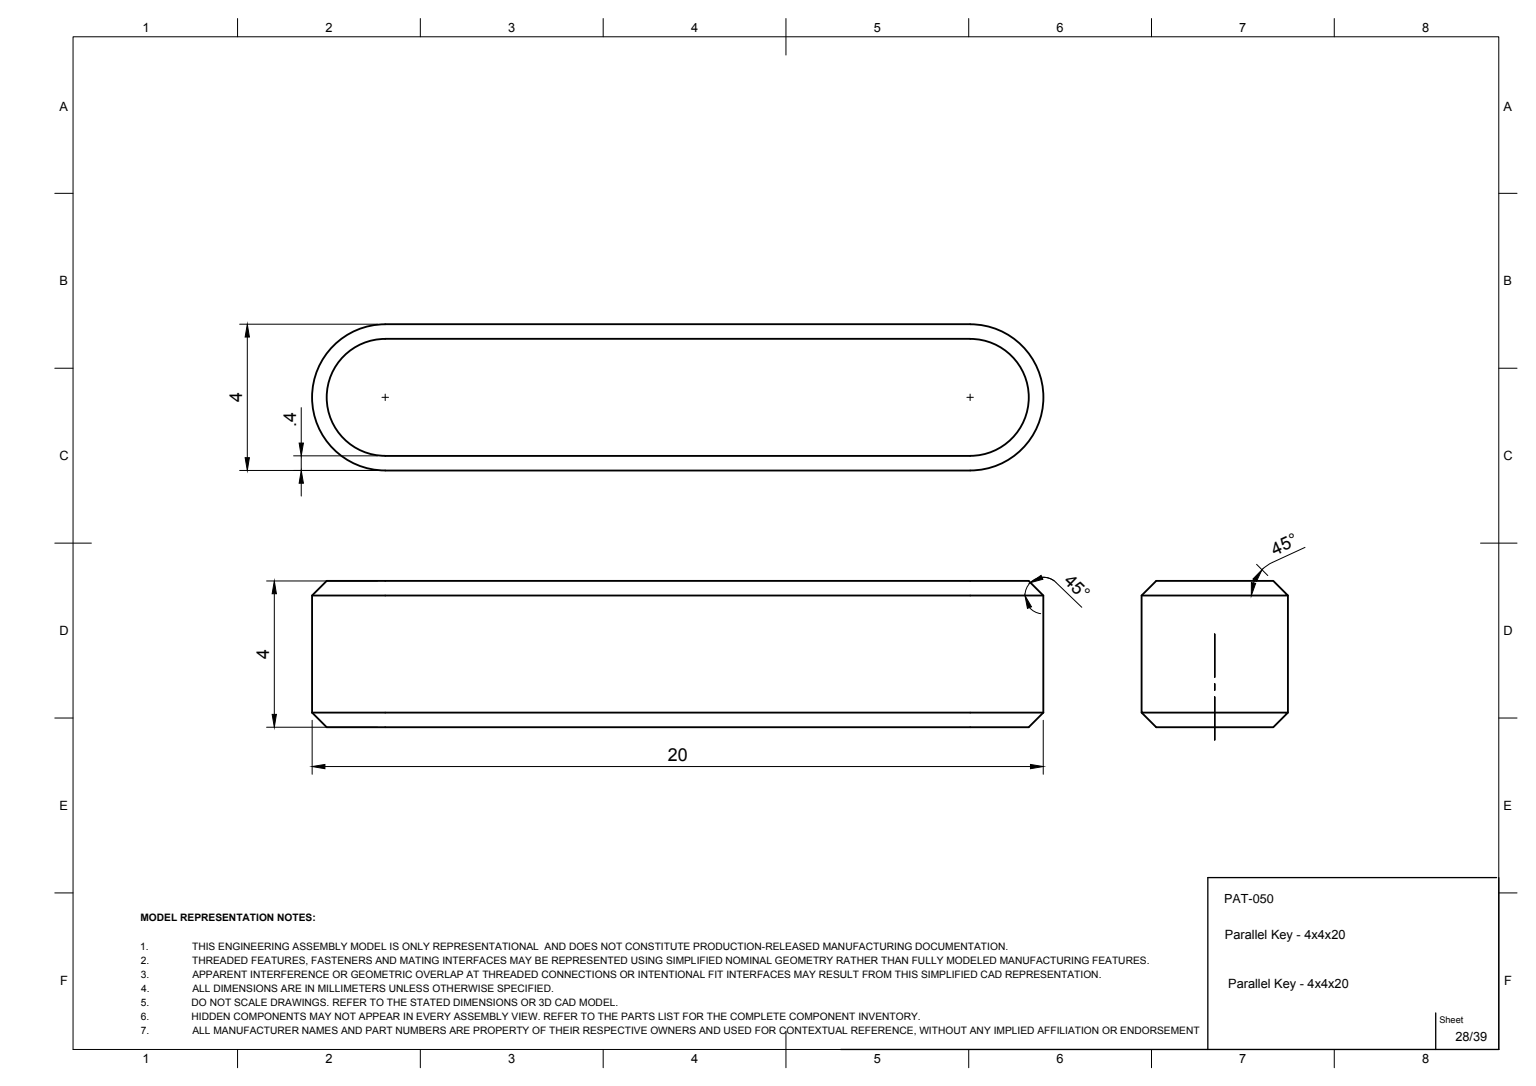
ISO-10303-21;
HEADER;
/* Generated by software containing ST-Developer
 * from STEP Tools, Inc. (www.steptools.com) 
 */

FILE_DESCRIPTION(
/* description */ ('Hand wheel with handle and shaft collar'),
/* implementation_level */ '2;1');

FILE_NAME(
/* name */ 'Parallel Key - 4x4x20.step',
/* time_stamp */ '2026-10-28T03:23:19-07:00',
/* author */ (''),
/* organization */ (''),
/* preprocessor_version */ 'ST-DEVELOPER v20.2',
/* originating_system */ 'Autodesk Translation Framework v15.17.0.0',
/* authorisation */ '');

FILE_SCHEMA (('AUTOMOTIVE_DESIGN { 1 0 10303 214 3 1 1 }'));
ENDSEC;

DATA;
#10=MECHANICAL_DESIGN_GEOMETRIC_PRESENTATION_REPRESENTATION('',(#423),#10510);
#308=CONICAL_SURFACE('',#6130,0.18,0.785398163397448);
#309=CONICAL_SURFACE('',#6134,0.18,0.785398163397448);
#310=CONICAL_SURFACE('',#6142,0.18,0.785398163397449);
#311=CONICAL_SURFACE('',#6145,0.18,0.785398163397449);
#352=SHAPE_REPRESENTATION_RELATIONSHIP('SRR','None',#10670,#384);
#384=ADVANCED_BREP_SHAPE_REPRESENTATION('',(#469),#10497);
#423=STYLED_ITEM('',(#10908),#469);
#469=MANIFOLD_SOLID_BREP('Body1',#5323);
#702=PLANE('',#6129);
#703=PLANE('',#6133);
#704=PLANE('',#6139);
#705=PLANE('',#6140);
#706=PLANE('',#6141);
#707=PLANE('',#6144);
#708=PLANE('',#6149);
#709=PLANE('',#6150);
#962=FACE_OUTER_BOUND('',#1376,.T.);
#963=FACE_OUTER_BOUND('',#1377,.T.);
#964=FACE_OUTER_BOUND('',#1378,.T.);
#965=FACE_OUTER_BOUND('',#1379,.T.);
#966=FACE_OUTER_BOUND('',#1380,.T.);
#967=FACE_OUTER_BOUND('',#1381,.T.);
#968=FACE_OUTER_BOUND('',#1382,.T.);
#969=FACE_OUTER_BOUND('',#1383,.T.);
#970=FACE_OUTER_BOUND('',#1384,.T.);
#971=FACE_OUTER_BOUND('',#1385,.T.);
#972=FACE_OUTER_BOUND('',#1386,.T.);
#973=FACE_OUTER_BOUND('',#1387,.T.);
#974=FACE_OUTER_BOUND('',#1388,.T.);
#975=FACE_OUTER_BOUND('',#1389,.T.);
#1376=EDGE_LOOP('',(#4407,#4408,#4409,#4410));
#1377=EDGE_LOOP('',(#4411,#4412,#4413,#4414));
#1378=EDGE_LOOP('',(#4415,#4416,#4417,#4418));
#1379=EDGE_LOOP('',(#4419,#4420,#4421,#4422));
#1380=EDGE_LOOP('',(#4423,#4424,#4425,#4426));
#1381=EDGE_LOOP('',(#4427,#4428,#4429,#4430));
#1382=EDGE_LOOP('',(#4431,#4432,#4433,#4434));
#1383=EDGE_LOOP('',(#4435,#4436,#4437,#4438));
#1384=EDGE_LOOP('',(#4439,#4440,#4441,#4442));
#1385=EDGE_LOOP('',(#4443,#4444,#4445,#4446));
#1386=EDGE_LOOP('',(#4447,#4448,#4449,#4450));
#1387=EDGE_LOOP('',(#4451,#4452,#4453,#4454));
#1388=EDGE_LOOP('',(#4455,#4456,#4457,#4458));
#1389=EDGE_LOOP('',(#4459,#4460,#4461,#4462));
#1714=LINE('',#9520,#2024);
#1715=LINE('',#9522,#2025);
#1716=LINE('',#9524,#2026);
#1717=LINE('',#9525,#2027);
#1718=LINE('',#9529,#2028);
#1719=LINE('',#9535,#2029);
#1720=LINE('',#9536,#2030);
#1721=LINE('',#9537,#2031);
#1722=LINE('',#9543,#2032);
#1723=LINE('',#9546,#2033);
#1724=LINE('',#9549,#2034);
#1725=LINE('',#9550,#2035);
#1726=LINE('',#9554,#2036);
#1727=LINE('',#9556,#2037);
#1728=LINE('',#9557,#2038);
#1729=LINE('',#9560,#2039);
#1730=LINE('',#9565,#2040);
#1731=LINE('',#9566,#2041);
#1732=LINE('',#9567,#2042);
#1733=LINE('',#9572,#2043);
#2024=VECTOR('',#7486,1.);
#2025=VECTOR('',#7487,1.);
#2026=VECTOR('',#7488,1.);
#2027=VECTOR('',#7489,1.);
#2028=VECTOR('',#7492,1.);
#2029=VECTOR('',#7499,1.);
#2030=VECTOR('',#7500,1.);
#2031=VECTOR('',#7501,1.);
#2032=VECTOR('',#7510,1.);
#2033=VECTOR('',#7513,1.);
#2034=VECTOR('',#7516,1.);
#2035=VECTOR('',#7517,1.);
#2036=VECTOR('',#7522,1.);
#2037=VECTOR('',#7523,1.);
#2038=VECTOR('',#7524,1.);
#2039=VECTOR('',#7527,1.);
#2040=VECTOR('',#7532,1.);
#2041=VECTOR('',#7533,1.);
#2042=VECTOR('',#7534,1.);
#2043=VECTOR('',#7543,1.);
#2335=CIRCLE('',#6131,0.16);
#2336=CIRCLE('',#6132,0.2);
#2337=CIRCLE('',#6135,0.16);
#2338=CIRCLE('',#6136,0.2);
#2339=CIRCLE('',#6138,0.2);
#2340=CIRCLE('',#6143,0.16);
#2341=CIRCLE('',#6146,0.2);
#2342=CIRCLE('',#6147,0.16);
#2735=VERTEX_POINT('',#9518);
#2736=VERTEX_POINT('',#9519);
#2737=VERTEX_POINT('',#9521);
#2738=VERTEX_POINT('',#9523);
#2739=VERTEX_POINT('',#9527);
#2740=VERTEX_POINT('',#9528);
#2741=VERTEX_POINT('',#9533);
#2742=VERTEX_POINT('',#9534);
#2743=VERTEX_POINT('',#9542);
#2744=VERTEX_POINT('',#9544);
#2745=VERTEX_POINT('',#9548);
#2746=VERTEX_POINT('',#9553);
#2747=VERTEX_POINT('',#9555);
#2748=VERTEX_POINT('',#9559);
#2749=VERTEX_POINT('',#9563);
#2750=VERTEX_POINT('',#9564);
#3321=EDGE_CURVE('',#2735,#2736,#1714,.T.);
#3322=EDGE_CURVE('',#2736,#2737,#1715,.T.);
#3323=EDGE_CURVE('',#2737,#2738,#1716,.T.);
#3324=EDGE_CURVE('',#2738,#2735,#1717,.T.);
#3325=EDGE_CURVE('',#2739,#2740,#1718,.T.);
#3326=EDGE_CURVE('',#2740,#2736,#2335,.T.);
#3327=EDGE_CURVE('',#2735,#2739,#2336,.T.);
#3328=EDGE_CURVE('',#2741,#2742,#1719,.T.);
#3329=EDGE_CURVE('',#2742,#2740,#1720,.T.);
#3330=EDGE_CURVE('',#2739,#2741,#1721,.T.);
#3331=EDGE_CURVE('',#2737,#2742,#2337,.T.);
#3332=EDGE_CURVE('',#2741,#2738,#2338,.T.);
#3333=EDGE_CURVE('',#2743,#2735,#1722,.T.);
#3334=EDGE_CURVE('',#2744,#2743,#2339,.T.);
#3335=EDGE_CURVE('',#2744,#2739,#1723,.T.);
#3336=EDGE_CURVE('',#2745,#2738,#1724,.T.);
#3337=EDGE_CURVE('',#2743,#2745,#1725,.T.);
#3338=EDGE_CURVE('',#2746,#2743,#1726,.T.);
#3339=EDGE_CURVE('',#2745,#2747,#1727,.T.);
#3340=EDGE_CURVE('',#2747,#2746,#1728,.T.);
#3341=EDGE_CURVE('',#2748,#2744,#1729,.T.);
#3342=EDGE_CURVE('',#2746,#2748,#2340,.T.);
#3343=EDGE_CURVE('',#2749,#2750,#1730,.T.);
#3344=EDGE_CURVE('',#2750,#2744,#1731,.T.);
#3345=EDGE_CURVE('',#2748,#2749,#1732,.T.);
#3346=EDGE_CURVE('',#2745,#2750,#2341,.T.);
#3347=EDGE_CURVE('',#2749,#2747,#2342,.T.);
#3348=EDGE_CURVE('',#2750,#2741,#1733,.T.);
#4407=ORIENTED_EDGE('',*,*,#3321,.T.);
#4408=ORIENTED_EDGE('',*,*,#3322,.T.);
#4409=ORIENTED_EDGE('',*,*,#3323,.T.);
#4410=ORIENTED_EDGE('',*,*,#3324,.T.);
#4411=ORIENTED_EDGE('',*,*,#3325,.T.);
#4412=ORIENTED_EDGE('',*,*,#3326,.T.);
#4413=ORIENTED_EDGE('',*,*,#3321,.F.);
#4414=ORIENTED_EDGE('',*,*,#3327,.T.);
#4415=ORIENTED_EDGE('',*,*,#3328,.T.);
#4416=ORIENTED_EDGE('',*,*,#3329,.T.);
#4417=ORIENTED_EDGE('',*,*,#3325,.F.);
#4418=ORIENTED_EDGE('',*,*,#3330,.T.);
#4419=ORIENTED_EDGE('',*,*,#3323,.F.);
#4420=ORIENTED_EDGE('',*,*,#3331,.T.);
#4421=ORIENTED_EDGE('',*,*,#3328,.F.);
#4422=ORIENTED_EDGE('',*,*,#3332,.T.);
#4423=ORIENTED_EDGE('',*,*,#3327,.F.);
#4424=ORIENTED_EDGE('',*,*,#3333,.F.);
#4425=ORIENTED_EDGE('',*,*,#3334,.F.);
#4426=ORIENTED_EDGE('',*,*,#3335,.T.);
#4427=ORIENTED_EDGE('',*,*,#3324,.F.);
#4428=ORIENTED_EDGE('',*,*,#3336,.F.);
#4429=ORIENTED_EDGE('',*,*,#3337,.F.);
#4430=ORIENTED_EDGE('',*,*,#3333,.T.);
#4431=ORIENTED_EDGE('',*,*,#3322,.F.);
#4432=ORIENTED_EDGE('',*,*,#3326,.F.);
#4433=ORIENTED_EDGE('',*,*,#3329,.F.);
#4434=ORIENTED_EDGE('',*,*,#3331,.F.);
#4435=ORIENTED_EDGE('',*,*,#3338,.T.);
#4436=ORIENTED_EDGE('',*,*,#3337,.T.);
#4437=ORIENTED_EDGE('',*,*,#3339,.T.);
#4438=ORIENTED_EDGE('',*,*,#3340,.T.);
#4439=ORIENTED_EDGE('',*,*,#3341,.T.);
#4440=ORIENTED_EDGE('',*,*,#3334,.T.);
#4441=ORIENTED_EDGE('',*,*,#3338,.F.);
#4442=ORIENTED_EDGE('',*,*,#3342,.T.);
#4443=ORIENTED_EDGE('',*,*,#3343,.T.);
#4444=ORIENTED_EDGE('',*,*,#3344,.T.);
#4445=ORIENTED_EDGE('',*,*,#3341,.F.);
#4446=ORIENTED_EDGE('',*,*,#3345,.T.);
#4447=ORIENTED_EDGE('',*,*,#3339,.F.);
#4448=ORIENTED_EDGE('',*,*,#3346,.T.);
#4449=ORIENTED_EDGE('',*,*,#3343,.F.);
#4450=ORIENTED_EDGE('',*,*,#3347,.T.);
#4451=ORIENTED_EDGE('',*,*,#3332,.F.);
#4452=ORIENTED_EDGE('',*,*,#3348,.F.);
#4453=ORIENTED_EDGE('',*,*,#3346,.F.);
#4454=ORIENTED_EDGE('',*,*,#3336,.T.);
#4455=ORIENTED_EDGE('',*,*,#3340,.F.);
#4456=ORIENTED_EDGE('',*,*,#3347,.F.);
#4457=ORIENTED_EDGE('',*,*,#3345,.F.);
#4458=ORIENTED_EDGE('',*,*,#3342,.F.);
#4459=ORIENTED_EDGE('',*,*,#3330,.F.);
#4460=ORIENTED_EDGE('',*,*,#3335,.F.);
#4461=ORIENTED_EDGE('',*,*,#3344,.F.);
#4462=ORIENTED_EDGE('',*,*,#3348,.T.);
#4951=CYLINDRICAL_SURFACE('',#6137,0.2);
#4952=CYLINDRICAL_SURFACE('',#6148,0.2);
#5174=ADVANCED_FACE('',(#962),#702,.T.);
#5175=ADVANCED_FACE('',(#963),#308,.T.);
#5176=ADVANCED_FACE('',(#964),#703,.T.);
#5177=ADVANCED_FACE('',(#965),#309,.T.);
#5178=ADVANCED_FACE('',(#966),#4951,.T.);
#5179=ADVANCED_FACE('',(#967),#704,.T.);
#5180=ADVANCED_FACE('',(#968),#705,.T.);
#5181=ADVANCED_FACE('',(#969),#706,.T.);
#5182=ADVANCED_FACE('',(#970),#310,.T.);
#5183=ADVANCED_FACE('',(#971),#707,.T.);
#5184=ADVANCED_FACE('',(#972),#311,.T.);
#5185=ADVANCED_FACE('',(#973),#4952,.T.);
#5186=ADVANCED_FACE('',(#974),#708,.F.);
#5187=ADVANCED_FACE('',(#975),#709,.T.);
#5323=CLOSED_SHELL('',(#5174,#5175,#5176,#5177,#5178,#5179,#5180,#5181,
#5182,#5183,#5184,#5185,#5186,#5187));
#6128=AXIS2_PLACEMENT_3D('',#9516,#7482,#7483);
#6129=AXIS2_PLACEMENT_3D('',#9517,#7484,#7485);
#6130=AXIS2_PLACEMENT_3D('',#9526,#7490,#7491);
#6131=AXIS2_PLACEMENT_3D('',#9530,#7493,#7494);
#6132=AXIS2_PLACEMENT_3D('',#9531,#7495,#7496);
#6133=AXIS2_PLACEMENT_3D('',#9532,#7497,#7498);
#6134=AXIS2_PLACEMENT_3D('',#9538,#7502,#7503);
#6135=AXIS2_PLACEMENT_3D('',#9539,#7504,#7505);
#6136=AXIS2_PLACEMENT_3D('',#9540,#7506,#7507);
#6137=AXIS2_PLACEMENT_3D('',#9541,#7508,#7509);
#6138=AXIS2_PLACEMENT_3D('',#9545,#7511,#7512);
#6139=AXIS2_PLACEMENT_3D('',#9547,#7514,#7515);
#6140=AXIS2_PLACEMENT_3D('',#9551,#7518,#7519);
#6141=AXIS2_PLACEMENT_3D('',#9552,#7520,#7521);
#6142=AXIS2_PLACEMENT_3D('',#9558,#7525,#7526);
#6143=AXIS2_PLACEMENT_3D('',#9561,#7528,#7529);
#6144=AXIS2_PLACEMENT_3D('',#9562,#7530,#7531);
#6145=AXIS2_PLACEMENT_3D('',#9568,#7535,#7536);
#6146=AXIS2_PLACEMENT_3D('',#9569,#7537,#7538);
#6147=AXIS2_PLACEMENT_3D('',#9570,#7539,#7540);
#6148=AXIS2_PLACEMENT_3D('',#9571,#7541,#7542);
#6149=AXIS2_PLACEMENT_3D('',#9573,#7544,#7545);
#6150=AXIS2_PLACEMENT_3D('',#9574,#7546,#7547);
#7482=DIRECTION('axis',(0.,0.,1.));
#7483=DIRECTION('refdir',(1.,0.,0.));
#7484=DIRECTION('center_axis',(0.,0.707106781186548,0.707106781186547));
#7485=DIRECTION('ref_axis',(1.,0.,0.));
#7486=DIRECTION('',(-1.96261557335472E-15,-0.707106781186547,0.707106781186548));
#7487=DIRECTION('',(1.,0.,0.));
#7488=DIRECTION('',(0.,0.707106781186547,-0.707106781186548));
#7489=DIRECTION('',(-1.,0.,0.));
#7490=DIRECTION('center_axis',(0.,0.,-1.));
#7491=DIRECTION('ref_axis',(0.,1.,0.));
#7492=DIRECTION('',(0.,0.707106781186548,0.707106781186548));
#7493=DIRECTION('center_axis',(0.,0.,-1.));
#7494=DIRECTION('ref_axis',(0.,1.,0.));
#7495=DIRECTION('center_axis',(0.,0.,1.));
#7496=DIRECTION('ref_axis',(0.,1.,0.));
#7497=DIRECTION('center_axis',(0.,-0.707106781186548,0.707106781186547));
#7498=DIRECTION('ref_axis',(1.,0.,0.));
#7499=DIRECTION('',(1.96261557335472E-15,0.707106781186547,0.707106781186548));
#7500=DIRECTION('',(-1.,0.,0.));
#7501=DIRECTION('',(1.,0.,0.));
#7502=DIRECTION('center_axis',(0.,0.,-1.));
#7503=DIRECTION('ref_axis',(0.,-1.,0.));
#7504=DIRECTION('center_axis',(0.,0.,-1.));
#7505=DIRECTION('ref_axis',(0.,-1.,0.));
#7506=DIRECTION('center_axis',(0.,0.,1.));
#7507=DIRECTION('ref_axis',(0.,-1.,0.));
#7508=DIRECTION('center_axis',(0.,0.,1.));
#7509=DIRECTION('ref_axis',(0.,1.,0.));
#7510=DIRECTION('',(0.,0.,1.));
#7511=DIRECTION('center_axis',(0.,0.,-1.));
#7512=DIRECTION('ref_axis',(0.,1.,0.));
#7513=DIRECTION('',(0.,0.,1.));
#7514=DIRECTION('center_axis',(0.,1.,0.));
#7515=DIRECTION('ref_axis',(-1.,0.,0.));
#7516=DIRECTION('',(0.,0.,1.));
#7517=DIRECTION('',(1.,0.,0.));
#7518=DIRECTION('center_axis',(0.,0.,1.));
#7519=DIRECTION('ref_axis',(1.,0.,0.));
#7520=DIRECTION('center_axis',(0.,0.707106781186548,-0.707106781186548));
#7521=DIRECTION('ref_axis',(-1.,0.,0.));
#7522=DIRECTION('',(1.96261557335472E-15,0.707106781186548,0.707106781186548));
#7523=DIRECTION('',(0.,-0.707106781186548,-0.707106781186548));
#7524=DIRECTION('',(-1.,0.,0.));
#7525=DIRECTION('center_axis',(0.,0.,1.));
#7526=DIRECTION('ref_axis',(0.,1.,0.));
#7527=DIRECTION('',(0.,-0.707106781186548,0.707106781186547));
#7528=DIRECTION('center_axis',(0.,0.,1.));
#7529=DIRECTION('ref_axis',(0.,1.,0.));
#7530=DIRECTION('center_axis',(0.,-0.707106781186548,-0.707106781186548));
#7531=DIRECTION('ref_axis',(-1.,0.,0.));
#7532=DIRECTION('',(-1.96261557335472E-15,-0.707106781186548,0.707106781186548));
#7533=DIRECTION('',(-1.,0.,0.));
#7534=DIRECTION('',(1.,0.,0.));
#7535=DIRECTION('center_axis',(0.,0.,1.));
#7536=DIRECTION('ref_axis',(0.,-1.,0.));
#7537=DIRECTION('center_axis',(0.,0.,-1.));
#7538=DIRECTION('ref_axis',(0.,-1.,0.));
#7539=DIRECTION('center_axis',(0.,0.,1.));
#7540=DIRECTION('ref_axis',(0.,-1.,0.));
#7541=DIRECTION('center_axis',(0.,0.,1.));
#7542=DIRECTION('ref_axis',(0.,-1.,0.));
#7543=DIRECTION('',(0.,0.,1.));
#7544=DIRECTION('center_axis',(0.,0.,1.));
#7545=DIRECTION('ref_axis',(1.,0.,0.));
#7546=DIRECTION('center_axis',(0.,-1.,0.));
#7547=DIRECTION('ref_axis',(1.,0.,0.));
#9516=CARTESIAN_POINT('',(0.,0.,0.));
#9517=CARTESIAN_POINT('Origin',(0.4,0.18,0.38));
#9518=CARTESIAN_POINT('',(-0.8,0.2,0.36));
#9519=CARTESIAN_POINT('',(-0.8,0.16,0.4));
#9520=CARTESIAN_POINT('',(-0.8,0.2,0.36));
#9521=CARTESIAN_POINT('',(0.8,0.16,0.4));
#9522=CARTESIAN_POINT('',(0.4,0.16,0.4));
#9523=CARTESIAN_POINT('',(0.8,0.2,0.36));
#9524=CARTESIAN_POINT('',(0.8,0.16,0.4));
#9525=CARTESIAN_POINT('',(0.4,0.2,0.36));
#9526=CARTESIAN_POINT('Origin',(-0.8,0.,0.38));
#9527=CARTESIAN_POINT('',(-0.8,-0.2,0.36));
#9528=CARTESIAN_POINT('',(-0.8,-0.16,0.4));
#9529=CARTESIAN_POINT('',(-0.8,-0.2,0.36));
#9530=CARTESIAN_POINT('Origin',(-0.8,0.,0.4));
#9531=CARTESIAN_POINT('Origin',(-0.8,0.,0.36));
#9532=CARTESIAN_POINT('Origin',(-0.4,-0.18,0.38));
#9533=CARTESIAN_POINT('',(0.8,-0.2,0.36));
#9534=CARTESIAN_POINT('',(0.8,-0.16,0.4));
#9535=CARTESIAN_POINT('',(0.8,-0.2,0.36));
#9536=CARTESIAN_POINT('',(-0.4,-0.16,0.4));
#9537=CARTESIAN_POINT('',(-0.4,-0.2,0.36));
#9538=CARTESIAN_POINT('Origin',(0.8,0.,0.38));
#9539=CARTESIAN_POINT('Origin',(0.8,0.,0.4));
#9540=CARTESIAN_POINT('Origin',(0.8,0.,0.36));
#9541=CARTESIAN_POINT('Origin',(-0.8,0.,0.));
#9542=CARTESIAN_POINT('',(-0.8,0.2,0.04));
#9543=CARTESIAN_POINT('',(-0.8,0.2,0.));
#9544=CARTESIAN_POINT('',(-0.8,-0.2,0.04));
#9545=CARTESIAN_POINT('Origin',(-0.8,0.,0.04));
#9546=CARTESIAN_POINT('',(-0.8,-0.2,0.));
#9547=CARTESIAN_POINT('Origin',(0.8,0.2,0.));
#9548=CARTESIAN_POINT('',(0.8,0.2,0.04));
#9549=CARTESIAN_POINT('',(0.8,0.2,0.));
#9550=CARTESIAN_POINT('',(0.4,0.2,0.04));
#9551=CARTESIAN_POINT('Origin',(0.,0.,0.4));
#9552=CARTESIAN_POINT('Origin',(0.4,0.18,0.02));
#9553=CARTESIAN_POINT('',(-0.8,0.16,0.));
#9554=CARTESIAN_POINT('',(-0.8,0.16,0.));
#9555=CARTESIAN_POINT('',(0.8,0.16,0.));
#9556=CARTESIAN_POINT('',(0.8,0.2,0.04));
#9557=CARTESIAN_POINT('',(0.4,0.16,0.));
#9558=CARTESIAN_POINT('Origin',(-0.8,0.,0.02));
#9559=CARTESIAN_POINT('',(-0.8,-0.16,0.));
#9560=CARTESIAN_POINT('',(-0.8,-0.16,0.));
#9561=CARTESIAN_POINT('Origin',(-0.8,0.,0.));
#9562=CARTESIAN_POINT('Origin',(-0.4,-0.18,0.02));
#9563=CARTESIAN_POINT('',(0.8,-0.16,0.));
#9564=CARTESIAN_POINT('',(0.8,-0.2,0.04));
#9565=CARTESIAN_POINT('',(0.8,-0.16,0.));
#9566=CARTESIAN_POINT('',(-0.4,-0.2,0.04));
#9567=CARTESIAN_POINT('',(-0.4,-0.16,0.));
#9568=CARTESIAN_POINT('Origin',(0.8,0.,0.02));
#9569=CARTESIAN_POINT('Origin',(0.8,0.,0.04));
#9570=CARTESIAN_POINT('Origin',(0.8,0.,0.));
#9571=CARTESIAN_POINT('Origin',(0.8,0.,0.));
#9572=CARTESIAN_POINT('',(0.8,-0.2,0.));
#9573=CARTESIAN_POINT('Origin',(0.,0.,0.));
#9574=CARTESIAN_POINT('Origin',(-0.8,-0.2,0.));
#10458=UNCERTAINTY_MEASURE_WITH_UNIT(LENGTH_MEASURE(0.001),#10511,
'DISTANCE_ACCURACY_VALUE',
'Maximum model space distance between geometric entities at asserted c
onnectivities');
#10471=UNCERTAINTY_MEASURE_WITH_UNIT(LENGTH_MEASURE(0.001),#10511,
'DISTANCE_ACCURACY_VALUE',
'Maximum model space distance between geometric entities at asserted c
onnectivities');
#10497=(
GEOMETRIC_REPRESENTATION_CONTEXT(3)
GLOBAL_UNCERTAINTY_ASSIGNED_CONTEXT((#10458))
GLOBAL_UNIT_ASSIGNED_CONTEXT((#10511,#10513,#10514))
REPRESENTATION_CONTEXT('','3D')
);
#10510=(
GEOMETRIC_REPRESENTATION_CONTEXT(3)
GLOBAL_UNCERTAINTY_ASSIGNED_CONTEXT((#10471))
GLOBAL_UNIT_ASSIGNED_CONTEXT((#10511,#10513,#10514))
REPRESENTATION_CONTEXT('','3D')
);
#10511=(
LENGTH_UNIT()
NAMED_UNIT(*)
SI_UNIT(.CENTI.,.METRE.)
);
#10513=(
NAMED_UNIT(*)
PLANE_ANGLE_UNIT()
SI_UNIT($,.RADIAN.)
);
#10514=(
NAMED_UNIT(*)
SI_UNIT($,.STERADIAN.)
SOLID_ANGLE_UNIT()
);
#10540=SHAPE_DEFINITION_REPRESENTATION(#10583,#10670);
#10583=PRODUCT_DEFINITION_SHAPE('',$,#10709);
#10670=SHAPE_REPRESENTATION('',(#6128),#10497);
#10683=PRODUCT_DEFINITION_CONTEXT('part definition',#10799,'design');
#10709=PRODUCT_DEFINITION('Parallel Key - 4x4x20',
'Parallel Key - 4x4x20',#10747,#10683);
#10747=PRODUCT_DEFINITION_FORMATION('',$,#10826);
#10799=APPLICATION_CONTEXT(
'Core Data for Automotive Mechanical Design Process');
#10800=PRODUCT_CONTEXT('part definition',#10799,'mechanical');
#10826=PRODUCT('Parallel Key - 4x4x20','Parallel Key - 4x4x20',
'Parallel Key - 4x4x20',(#10800));
#10902=COLOUR_RGB('Grey',0.48,0.52,0.57);
#10903=FILL_AREA_STYLE_COLOUR('',#10902);
#10904=FILL_AREA_STYLE('',(#10903));
#10905=SURFACE_STYLE_FILL_AREA(#10904);
#10906=SURFACE_SIDE_STYLE('',(#10905));
#10907=SURFACE_STYLE_USAGE(.BOTH.,#10906);
#10908=PRESENTATION_STYLE_ASSIGNMENT((#10907));
ENDSEC;
END-ISO-10303-21;
